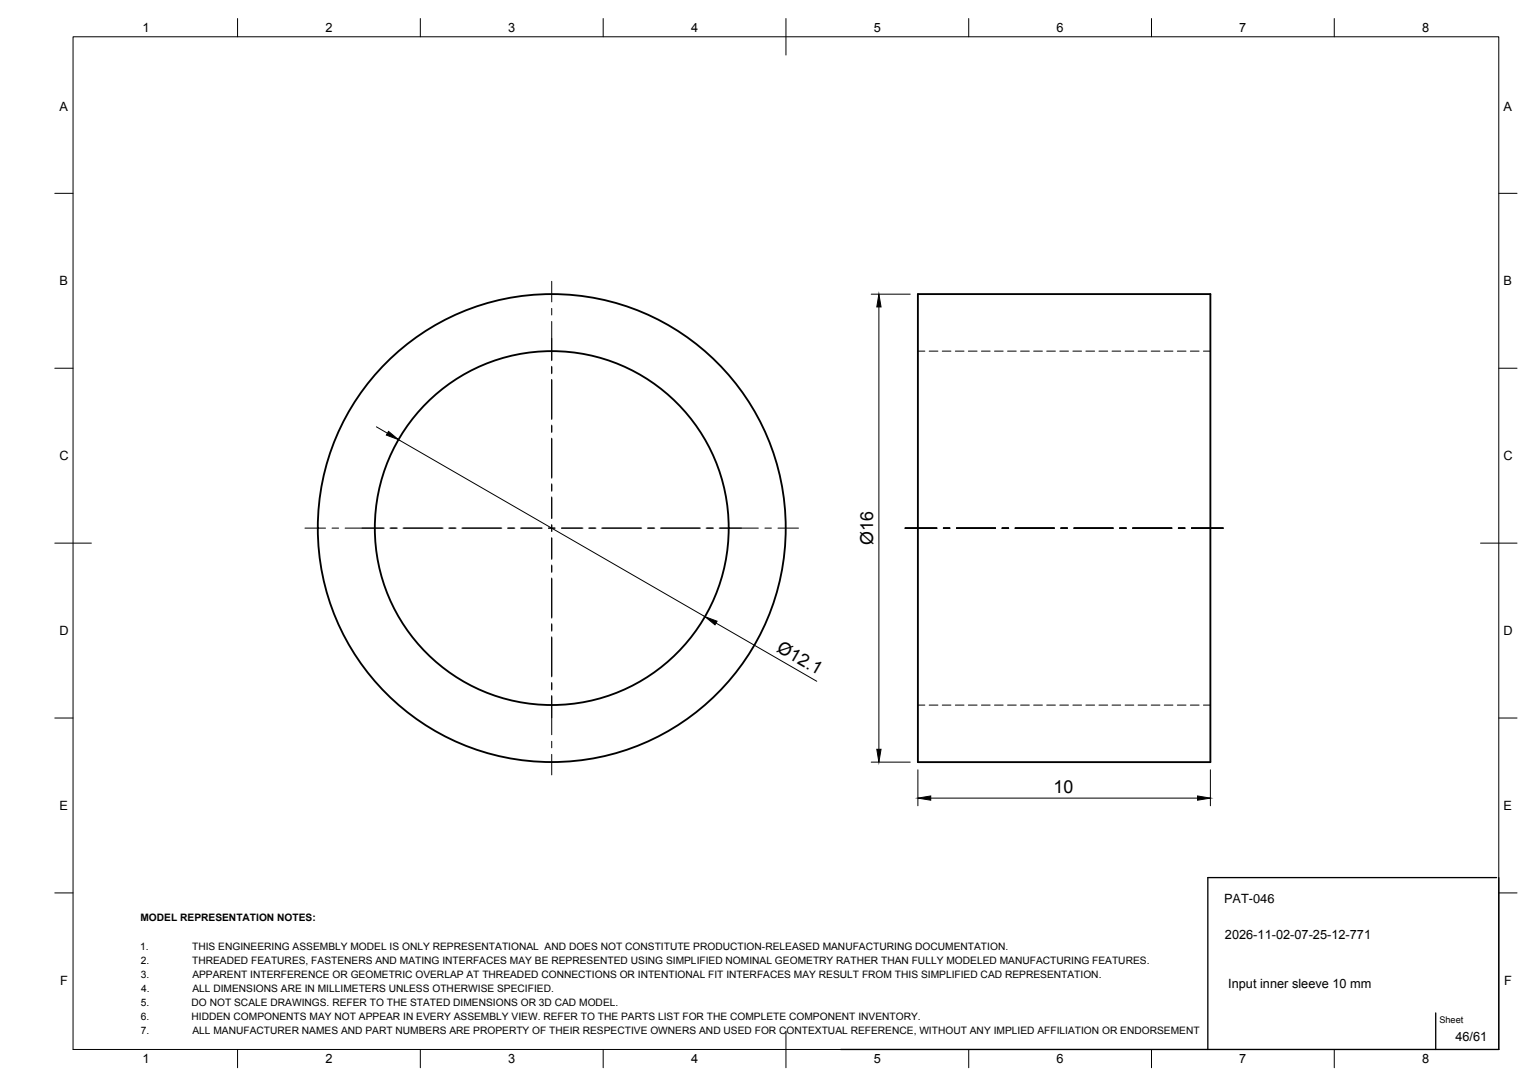
ISO-10303-21;
HEADER;
/* Generated by software containing ST-Developer
 * from STEP Tools, Inc. (www.steptools.com) 
 */

FILE_DESCRIPTION(
/* description */ ('Gear mesh backlash fixture'),
/* implementation_level */ '2;1');

FILE_NAME(
/* name */ 'Input inner sleeve 10 mm.step',
/* time_stamp */ '2026-10-28T03:26:00-07:00',
/* author */ (''),
/* organization */ (''),
/* preprocessor_version */ 'ST-DEVELOPER v20.2',
/* originating_system */ 'Autodesk Translation Framework v15.17.0.0',
/* authorisation */ '');

FILE_SCHEMA (('AUTOMOTIVE_DESIGN { 1 0 10303 214 3 1 1 }'));
ENDSEC;

DATA;
#10=MECHANICAL_DESIGN_GEOMETRIC_PRESENTATION_REPRESENTATION('',(#1065),#57900);
#950=SHAPE_REPRESENTATION_RELATIONSHIP('SRR','None',#58150,#1000);
#1000=ADVANCED_BREP_SHAPE_REPRESENTATION('',(#1128),#57883);
#1065=STYLED_ITEM('',(#58458),#1128);
#1128=MANIFOLD_SOLID_BREP('Body1',#13627);
#1295=FACE_BOUND('',#3029,.T.);
#1296=FACE_BOUND('',#3031,.T.);
#1559=PLANE('',#15074);
#1560=PLANE('',#15075);
#2109=FACE_OUTER_BOUND('',#3026,.T.);
#2110=FACE_OUTER_BOUND('',#3027,.T.);
#2111=FACE_OUTER_BOUND('',#3028,.T.);
#2112=FACE_OUTER_BOUND('',#3030,.T.);
#3026=EDGE_LOOP('',(#10735,#10736,#10737,#10738));
#3027=EDGE_LOOP('',(#10739,#10740,#10741,#10742));
#3028=EDGE_LOOP('',(#10743));
#3029=EDGE_LOOP('',(#10744));
#3030=EDGE_LOOP('',(#10745));
#3031=EDGE_LOOP('',(#10746));
#3893=LINE('',#22059,#4782);
#3894=LINE('',#22065,#4783);
#4782=VECTOR('',#17810,0.605);
#4783=VECTOR('',#17817,0.8);
#5592=CIRCLE('',#15069,0.605);
#5593=CIRCLE('',#15070,0.605);
#5594=CIRCLE('',#15072,0.8);
#5595=CIRCLE('',#15073,0.8);
#6410=VERTEX_POINT('',#22056);
#6411=VERTEX_POINT('',#22058);
#6412=VERTEX_POINT('',#22062);
#6413=VERTEX_POINT('',#22064);
#7954=EDGE_CURVE('',#6410,#6410,#5592,.T.);
#7955=EDGE_CURVE('',#6410,#6411,#3893,.T.);
#7956=EDGE_CURVE('',#6411,#6411,#5593,.T.);
#7957=EDGE_CURVE('',#6412,#6412,#5594,.T.);
#7958=EDGE_CURVE('',#6412,#6413,#3894,.T.);
#7959=EDGE_CURVE('',#6413,#6413,#5595,.T.);
#10735=ORIENTED_EDGE('',*,*,#7954,.F.);
#10736=ORIENTED_EDGE('',*,*,#7955,.T.);
#10737=ORIENTED_EDGE('',*,*,#7956,.T.);
#10738=ORIENTED_EDGE('',*,*,#7955,.F.);
#10739=ORIENTED_EDGE('',*,*,#7957,.F.);
#10740=ORIENTED_EDGE('',*,*,#7958,.T.);
#10741=ORIENTED_EDGE('',*,*,#7959,.T.);
#10742=ORIENTED_EDGE('',*,*,#7958,.F.);
#10743=ORIENTED_EDGE('',*,*,#7957,.T.);
#10744=ORIENTED_EDGE('',*,*,#7954,.T.);
#10745=ORIENTED_EDGE('',*,*,#7959,.F.);
#10746=ORIENTED_EDGE('',*,*,#7956,.F.);
#12720=CYLINDRICAL_SURFACE('',#15068,0.605);
#12721=CYLINDRICAL_SURFACE('',#15071,0.8);
#13226=ADVANCED_FACE('',(#2109),#12720,.F.);
#13227=ADVANCED_FACE('',(#2110),#12721,.T.);
#13228=ADVANCED_FACE('',(#2111,#1295),#1559,.T.);
#13229=ADVANCED_FACE('',(#2112,#1296),#1560,.F.);
#13627=CLOSED_SHELL('',(#13226,#13227,#13228,#13229));
#15067=AXIS2_PLACEMENT_3D('',#22054,#17804,#17805);
#15068=AXIS2_PLACEMENT_3D('',#22055,#17806,#17807);
#15069=AXIS2_PLACEMENT_3D('',#22057,#17808,#17809);
#15070=AXIS2_PLACEMENT_3D('',#22060,#17811,#17812);
#15071=AXIS2_PLACEMENT_3D('',#22061,#17813,#17814);
#15072=AXIS2_PLACEMENT_3D('',#22063,#17815,#17816);
#15073=AXIS2_PLACEMENT_3D('',#22066,#17818,#17819);
#15074=AXIS2_PLACEMENT_3D('',#22067,#17820,#17821);
#15075=AXIS2_PLACEMENT_3D('',#22068,#17822,#17823);
#17804=DIRECTION('axis',(0.,0.,1.));
#17805=DIRECTION('refdir',(1.,0.,0.));
#17806=DIRECTION('center_axis',(0.,0.,1.));
#17807=DIRECTION('ref_axis',(1.,0.,0.));
#17808=DIRECTION('center_axis',(0.,0.,-1.));
#17809=DIRECTION('ref_axis',(1.,0.,0.));
#17810=DIRECTION('',(0.,0.,-1.));
#17811=DIRECTION('center_axis',(0.,0.,-1.));
#17812=DIRECTION('ref_axis',(1.,0.,0.));
#17813=DIRECTION('center_axis',(0.,0.,1.));
#17814=DIRECTION('ref_axis',(1.,0.,0.));
#17815=DIRECTION('center_axis',(0.,0.,1.));
#17816=DIRECTION('ref_axis',(1.,0.,0.));
#17817=DIRECTION('',(0.,0.,-1.));
#17818=DIRECTION('center_axis',(0.,0.,1.));
#17819=DIRECTION('ref_axis',(1.,0.,0.));
#17820=DIRECTION('center_axis',(0.,0.,1.));
#17821=DIRECTION('ref_axis',(1.,0.,0.));
#17822=DIRECTION('center_axis',(0.,0.,1.));
#17823=DIRECTION('ref_axis',(1.,0.,0.));
#22054=CARTESIAN_POINT('',(0.,0.,0.));
#22055=CARTESIAN_POINT('Origin',(0.,0.,7.));
#22056=CARTESIAN_POINT('',(-0.605,-7.40911313484149E-17,8.));
#22057=CARTESIAN_POINT('Origin',(0.,0.,8.));
#22058=CARTESIAN_POINT('',(-0.605,-7.40911313484149E-17,7.));
#22059=CARTESIAN_POINT('',(-0.605,-7.40911313484149E-17,7.));
#22060=CARTESIAN_POINT('Origin',(0.,0.,7.));
#22061=CARTESIAN_POINT('Origin',(0.,0.,7.));
#22062=CARTESIAN_POINT('',(-0.8,-9.79717439317883E-17,8.));
#22063=CARTESIAN_POINT('Origin',(0.,0.,8.));
#22064=CARTESIAN_POINT('',(-0.8,-9.79717439317883E-17,7.));
#22065=CARTESIAN_POINT('',(-0.8,-9.79717439317883E-17,7.));
#22066=CARTESIAN_POINT('Origin',(0.,0.,7.));
#22067=CARTESIAN_POINT('Origin',(0.,0.,8.));
#22068=CARTESIAN_POINT('Origin',(0.,0.,7.));
#57824=UNCERTAINTY_MEASURE_WITH_UNIT(LENGTH_MEASURE(0.001),#57901,
'DISTANCE_ACCURACY_VALUE',
'Maximum model space distance between geometric entities at asserted c
onnectivities');
#57841=UNCERTAINTY_MEASURE_WITH_UNIT(LENGTH_MEASURE(0.001),#57901,
'DISTANCE_ACCURACY_VALUE',
'Maximum model space distance between geometric entities at asserted c
onnectivities');
#57883=(
GEOMETRIC_REPRESENTATION_CONTEXT(3)
GLOBAL_UNCERTAINTY_ASSIGNED_CONTEXT((#57824))
GLOBAL_UNIT_ASSIGNED_CONTEXT((#57901,#57903,#57904))
REPRESENTATION_CONTEXT('','3D')
);
#57900=(
GEOMETRIC_REPRESENTATION_CONTEXT(3)
GLOBAL_UNCERTAINTY_ASSIGNED_CONTEXT((#57841))
GLOBAL_UNIT_ASSIGNED_CONTEXT((#57901,#57903,#57904))
REPRESENTATION_CONTEXT('','3D')
);
#57901=(
LENGTH_UNIT()
NAMED_UNIT(*)
SI_UNIT(.CENTI.,.METRE.)
);
#57903=(
NAMED_UNIT(*)
PLANE_ANGLE_UNIT()
SI_UNIT($,.RADIAN.)
);
#57904=(
NAMED_UNIT(*)
SI_UNIT($,.STERADIAN.)
SOLID_ANGLE_UNIT()
);
#57946=SHAPE_DEFINITION_REPRESENTATION(#58017,#58150);
#58017=PRODUCT_DEFINITION_SHAPE('',$,#58209);
#58150=SHAPE_REPRESENTATION('',(#15067),#57883);
#58167=PRODUCT_DEFINITION_CONTEXT('part definition',#58343,'design');
#58209=PRODUCT_DEFINITION('Input inner sleeve 10 mm',
'Input inner sleeve 10 mm',#58267,#58167);
#58267=PRODUCT_DEFINITION_FORMATION('',$,#58386);
#58343=APPLICATION_CONTEXT(
'Core Data for Automotive Mechanical Design Process');
#58344=PRODUCT_CONTEXT('part definition',#58343,'mechanical');
#58386=PRODUCT('Input inner sleeve 10 mm','Input inner sleeve 10 mm',
'Input inner sleeve 10 mm',(#58344));
#58452=COLOUR_RGB('Sky Blue',0.24,0.69,0.87);
#58453=FILL_AREA_STYLE_COLOUR('',#58452);
#58454=FILL_AREA_STYLE('',(#58453));
#58455=SURFACE_STYLE_FILL_AREA(#58454);
#58456=SURFACE_SIDE_STYLE('',(#58455));
#58457=SURFACE_STYLE_USAGE(.BOTH.,#58456);
#58458=PRESENTATION_STYLE_ASSIGNMENT((#58457));
ENDSEC;
END-ISO-10303-21;
